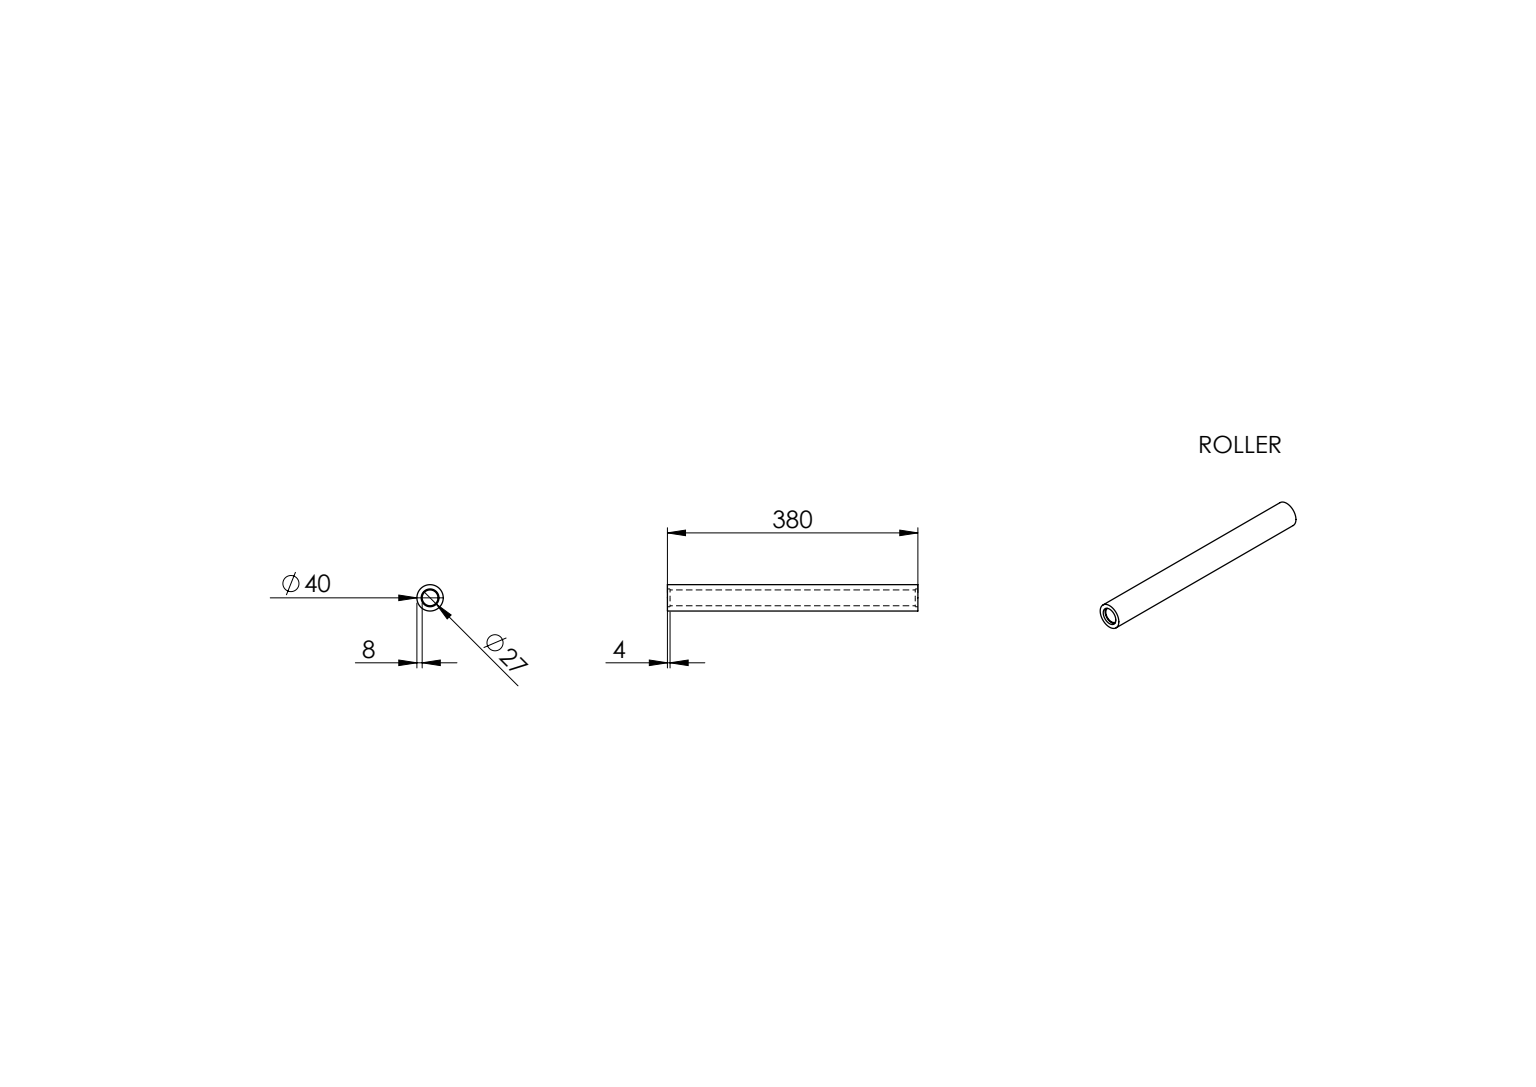
ISO-10303-21;
HEADER;
FILE_DESCRIPTION (('STEP AP214'),
    '1' );
FILE_NAME ('roller.step',
    '2026-10-24T13:33:06',
    ( '' ),
    ( '' ),
    'SwSTEP 2.0',
    'SolidWorks 2026',
    '' );
FILE_SCHEMA (( 'AUTOMOTIVE_DESIGN' ));
ENDSEC;

DATA;
#56=DIRECTION ( 'NONE',  ( 1.000000000000000000, 0.000000000000000000, 0.000000000000000000 ) ) ;
#77=FACE_OUTER_BOUND ( 'NONE', #3479, .T. ) ;
#137=ORIENTED_EDGE ( 'NONE', *, *, #8244, .F. ) ;
#171=CIRCLE ( 'NONE', #3238, 20.00000000000000000 ) ;
#191=VERTEX_POINT ( 'NONE', #7546 ) ;
#269=LINE ( 'NONE', #13422, #9164 ) ;
#370=DIRECTION ( 'NONE',  ( -1.000000000000000000, 0.000000000000000000, 0.000000000000000000 ) ) ;
#456=ORIENTED_EDGE ( 'NONE', *, *, #9949, .T. ) ;
#491=( GEOMETRIC_REPRESENTATION_CONTEXT ( 3 ) GLOBAL_UNCERTAINTY_ASSIGNED_CONTEXT ( ( #7550 ) ) GLOBAL_UNIT_ASSIGNED_CONTEXT ( ( #9395, #10194, #4976 ) ) REPRESENTATION_CONTEXT ( 'NONE', 'WORKASPACE' ) );
#495=EDGE_LOOP ( 'NONE', ( #2805, #3128, #6532, #2703 ) ) ;
#498=VERTEX_POINT ( 'NONE', #10666 ) ;
#571=DIRECTION ( 'NONE',  ( -0.000000000000000000, -0.000000000000000000, -1.000000000000000000 ) ) ;
#599=CARTESIAN_POINT ( 'NONE',  ( 0.000000000000000000, 0.000000000000000000, 186.0000000000000000 ) ) ;
#655=CARTESIAN_POINT ( 'NONE',  ( 0.000000000000000000, 0.000000000000000000, 186.0000000000000000 ) ) ;
#810=DIRECTION ( 'NONE',  ( 1.000000000000000000, 0.000000000000000000, 0.000000000000000000 ) ) ;
#928=CIRCLE ( 'NONE', #9057, 13.50000000000000000 ) ;
#944=ORIENTED_EDGE ( 'NONE', *, *, #12577, .T. ) ;
#1054=ADVANCED_BREP_SHAPE_REPRESENTATION ( '', ( #8362, #14039 ), #4925 ) ;
#1097=AXIS2_PLACEMENT_3D ( 'NONE', #1465, #6917, #7059 ) ;
#1124=AXIS2_PLACEMENT_3D ( 'NONE', #13971, #12956, #3031 ) ;
#1240=DIRECTION ( 'NONE',  ( 0.000000000000000000, 0.000000000000000000, 1.000000000000000000 ) ) ;
#1273=CARTESIAN_POINT ( 'NONE',  ( -13.50000000000000000, 1.653273178848926867E-15, 186.0000000000000000 ) ) ;
#1296=ORIENTED_EDGE ( 'NONE', *, *, #6936, .T. ) ;
#1318=AXIS2_PLACEMENT_3D ( 'NONE', #6760, #2269, #6696 ) ;
#1331=EDGE_CURVE ( 'NONE', #11674, #5306, #12710, .T. ) ;
#1464=FACE_OUTER_BOUND ( 'NONE', #495, .T. ) ;
#1465=CARTESIAN_POINT ( 'NONE',  ( 0.000000000000000000, 0.000000000000000000, 190.0000000000000000 ) ) ;
#1505=EDGE_LOOP ( 'NONE', ( #3985, #10939 ) ) ;
#1537=CARTESIAN_POINT ( 'NONE',  ( 0.000000000000000000, 0.000000000000000000, -186.0000000000000000 ) ) ;
#1589=( LENGTH_UNIT ( ) NAMED_UNIT ( * ) SI_UNIT ( .MILLI., .METRE. ) );
#1620=SURFACE_STYLE_FILL_AREA ( #2512 ) ;
#1624=CARTESIAN_POINT ( 'NONE',  ( 0.000000000000000000, 0.000000000000000000, -186.0000000000000000 ) ) ;
#1684=UNCERTAINTY_MEASURE_WITH_UNIT (LENGTH_MEASURE( 1.000000000000000082E-05 ), #1589, 'distance_accuracy_value', 'NONE');
#1739=PRODUCT_CONTEXT ( 'NONE', #11106, 'mechanical' ) ;
#1792=ADVANCED_FACE ( 'NONE', ( #5012 ), #10742, .F. ) ;
#1814=( NAMED_UNIT ( * ) PLANE_ANGLE_UNIT ( ) SI_UNIT ( $, .RADIAN. ) );
#1924=APPLICATION_CONTEXT ( 'automotive_design' ) ;
#1936=EDGE_LOOP ( 'NONE', ( #2189, #10105 ) ) ;
#1948=EDGE_CURVE ( 'NONE', #3491, #8933, #13191, .T. ) ;
#1979=CARTESIAN_POINT ( 'NONE',  ( 12.00000000000000000, 1.469576158976823947E-15, 186.0000000000000000 ) ) ;
#2027=AXIS2_PLACEMENT_3D ( 'NONE', #10148, #6674, #12325 ) ;
#2063=CYLINDRICAL_SURFACE ( 'NONE', #8959, 13.50000000000000000 ) ;
#2070=CIRCLE ( 'NONE', #12034, 13.50000000000000000 ) ;
#2075=ORIENTED_EDGE ( 'NONE', *, *, #12736, .F. ) ;
#2081=AXIS2_PLACEMENT_3D ( 'NONE', #6577, #11081, #6714 ) ;
#2151=EDGE_CURVE ( 'NONE', #4585, #8933, #7405, .T. ) ;
#2189=ORIENTED_EDGE ( 'NONE', *, *, #13813, .F. ) ;
#2217=ADVANCED_FACE ( 'NONE', ( #13247, #6644 ), #8752, .T. ) ;
#2269=DIRECTION ( 'NONE',  ( 0.000000000000000000, 0.000000000000000000, 1.000000000000000000 ) ) ;
#2309=DIRECTION ( 'NONE',  ( -0.000000000000000000, -0.000000000000000000, 1.000000000000000000 ) ) ;
#2414=DIRECTION ( 'NONE',  ( 1.000000000000000000, 0.000000000000000000, 0.000000000000000000 ) ) ;
#2437=VERTEX_POINT ( 'NONE', #8958 ) ;
#2460=DIRECTION ( 'NONE',  ( 0.000000000000000000, 0.000000000000000000, 1.000000000000000000 ) ) ;
#2512=FILL_AREA_STYLE ('',( #5766 ) ) ;
#2703=ORIENTED_EDGE ( 'NONE', *, *, #3672, .T. ) ;
#2712=ORIENTED_EDGE ( 'NONE', *, *, #6511, .T. ) ;
#2727=SHAPE_REPRESENTATION_RELATIONSHIP ( 'NONE' , 'NONE' ,  #11637, #1054 ) ;
#2755=ORIENTED_EDGE ( 'NONE', *, *, #4202, .T. ) ;
#2759=ORIENTED_EDGE ( 'NONE', *, *, #3672, .F. ) ;
#2783=CARTESIAN_POINT ( 'NONE',  ( -13.50000000000000000, 0.000000000000000000, -186.0000000000000000 ) ) ;
#2794=CARTESIAN_POINT ( 'NONE',  ( -13.50000000000000000, 0.000000000000000000, -190.0000000000000000 ) ) ;
#2805=ORIENTED_EDGE ( 'NONE', *, *, #11204, .F. ) ;
#2810=VECTOR ( 'NONE', #7862, 1000.000000000000000 ) ;
#2822=( NAMED_UNIT ( * ) PLANE_ANGLE_UNIT ( ) SI_UNIT ( $, .RADIAN. ) );
#2862=CYLINDRICAL_SURFACE ( 'NONE', #13359, 13.50000000000000000 ) ;
#2866=DIRECTION ( 'NONE',  ( 0.000000000000000000, 0.000000000000000000, -1.000000000000000000 ) ) ;
#2910=CARTESIAN_POINT ( 'NONE',  ( -20.00000000000000000, 0.000000000000000000, -190.0000000000000000 ) ) ;
#3006=FACE_BOUND ( 'NONE', #5352, .T. ) ;
#3031=DIRECTION ( 'NONE',  ( -1.000000000000000000, 0.000000000000000000, 0.000000000000000000 ) ) ;
#3101=FACE_OUTER_BOUND ( 'NONE', #12272, .T. ) ;
#3107=DIRECTION ( 'NONE',  ( 1.000000000000000000, 0.000000000000000000, 0.000000000000000000 ) ) ;
#3119=CARTESIAN_POINT ( 'NONE',  ( -20.00000000000000000, 0.000000000000000000, 190.0000000000000000 ) ) ;
#3128=ORIENTED_EDGE ( 'NONE', *, *, #4828, .F. ) ;
#3226=CARTESIAN_POINT ( 'NONE',  ( 0.000000000000000000, 0.000000000000000000, 190.0000000000000000 ) ) ;
#3238=AXIS2_PLACEMENT_3D ( 'NONE', #7957, #2460, #6956 ) ;
#3276=CARTESIAN_POINT ( 'NONE',  ( 20.00000000000000000, 2.449293598294706513E-15, 190.0000000000000000 ) ) ;
#3357=ADVANCED_FACE ( 'NONE', ( #77 ), #5296, .F. ) ;
#3367=FACE_OUTER_BOUND ( 'NONE', #7390, .T. ) ;
#3479=EDGE_LOOP ( 'NONE', ( #3545, #1296, #9689, #9133 ) ) ;
#3491=VERTEX_POINT ( 'NONE', #9320 ) ;
#3512=CARTESIAN_POINT ( 'NONE',  ( 0.000000000000000000, 0.000000000000000000, 186.0000000000000000 ) ) ;
#3520=DIRECTION ( 'NONE',  ( 1.000000000000000000, 0.000000000000000000, 0.000000000000000000 ) ) ;
#3539=ADVANCED_FACE ( 'NONE', ( #11426 ), #6123, .T. ) ;
#3545=ORIENTED_EDGE ( 'NONE', *, *, #5646, .T. ) ;
#3555=DIRECTION ( 'NONE',  ( -1.000000000000000000, 0.000000000000000000, 0.000000000000000000 ) ) ;
#3571=DIRECTION ( 'NONE',  ( 1.000000000000000000, 0.000000000000000000, 0.000000000000000000 ) ) ;
#3581=VERTEX_POINT ( 'NONE', #1979 ) ;
#3622=FACE_OUTER_BOUND ( 'NONE', #11623, .T. ) ;
#3642=CIRCLE ( 'NONE', #1318, 20.00000000000000000 ) ;
#3672=EDGE_CURVE ( 'NONE', #191, #8653, #928, .T. ) ;
#3744=AXIS2_PLACEMENT_3D ( 'NONE', #5000, #13836, #6082 ) ;
#3761=ORIENTED_EDGE ( 'NONE', *, *, #5646, .F. ) ;
#3785=ORIENTED_EDGE ( 'NONE', *, *, #12600, .F. ) ;
#3841=CARTESIAN_POINT ( 'NONE',  ( 0.000000000000000000, 0.000000000000000000, 190.0000000000000000 ) ) ;
#3885=ORIENTED_EDGE ( 'NONE', *, *, #6936, .F. ) ;
#3927=DIRECTION ( 'NONE',  ( 0.000000000000000000, 0.000000000000000000, 1.000000000000000000 ) ) ;
#3935=AXIS2_PLACEMENT_3D ( 'NONE', #7654, #9770, #12149 ) ;
#3952=DIRECTION ( 'NONE',  ( -0.000000000000000000, -0.000000000000000000, -1.000000000000000000 ) ) ;
#3985=ORIENTED_EDGE ( 'NONE', *, *, #8012, .F. ) ;
#4003=STYLED_ITEM ( 'NONE', ( #12442 ), #1054 ) ;
#4123=CIRCLE ( 'NONE', #5473, 20.00000000000000000 ) ;
#4195=EDGE_LOOP ( 'NONE', ( #2759, #5420 ) ) ;
#4202=EDGE_CURVE ( 'NONE', #8845, #7342, #171, .T. ) ;
#4203=ADVANCED_FACE ( 'NONE', ( #3622 ), #10363, .T. ) ;
#4210=CARTESIAN_POINT ( 'NONE',  ( -12.00000000000000000, 0.000000000000000000, 190.0000000000000000 ) ) ;
#4380=ORIENTED_EDGE ( 'NONE', *, *, #9949, .F. ) ;
#4448=LINE ( 'NONE', #8868, #13591 ) ;
#4513=ORIENTED_EDGE ( 'NONE', *, *, #11633, .T. ) ;
#4516=FACE_BOUND ( 'NONE', #1505, .T. ) ;
#4567=CARTESIAN_POINT ( 'NONE',  ( 0.000000000000000000, 0.000000000000000000, 186.0000000000000000 ) ) ;
#4585=VERTEX_POINT ( 'NONE', #10949 ) ;
#4644=VECTOR ( 'NONE', #13052, 1000.000000000000000 ) ;
#4647=CARTESIAN_POINT ( 'NONE',  ( 20.00000000000000000, 2.449293598294706513E-15, -190.0000000000000000 ) ) ;
#4755=DIRECTION ( 'NONE',  ( -1.000000000000000000, 0.000000000000000000, 0.000000000000000000 ) ) ;
#4762=FACE_OUTER_BOUND ( 'NONE', #8447, .T. ) ;
#4783=CYLINDRICAL_SURFACE ( 'NONE', #6286, 13.50000000000000000 ) ;
#4804=DIRECTION ( 'NONE',  ( -0.000000000000000000, -0.000000000000000000, 1.000000000000000000 ) ) ;
#4816=CIRCLE ( 'NONE', #2027, 13.50000000000000000 ) ;
#4828=EDGE_CURVE ( 'NONE', #2437, #12064, #2070, .T. ) ;
#4878=ORIENTED_EDGE ( 'NONE', *, *, #11204, .T. ) ;
#4925=( GEOMETRIC_REPRESENTATION_CONTEXT ( 3 ) GLOBAL_UNCERTAINTY_ASSIGNED_CONTEXT ( ( #11924 ) ) GLOBAL_UNIT_ASSIGNED_CONTEXT ( ( #8462, #2822, #9489 ) ) REPRESENTATION_CONTEXT ( 'NONE', 'WORKASPACE' ) );
#4976=( NAMED_UNIT ( * ) SI_UNIT ( $, .STERADIAN. ) SOLID_ANGLE_UNIT ( ) );
#4992=EDGE_CURVE ( 'NONE', #498, #11674, #12043, .T. ) ;
#5000=CARTESIAN_POINT ( 'NONE',  ( 0.000000000000000000, 0.000000000000000000, 186.0000000000000000 ) ) ;
#5012=FACE_OUTER_BOUND ( 'NONE', #13790, .T. ) ;
#5048=AXIS2_PLACEMENT_3D ( 'NONE', #12411, #4804, #3571 ) ;
#5077=DIRECTION ( 'NONE',  ( 1.000000000000000000, 0.000000000000000000, 0.000000000000000000 ) ) ;
#5296=CYLINDRICAL_SURFACE ( 'NONE', #6955, 12.00000000000000000 ) ;
#5299=AXIS2_PLACEMENT_3D ( 'NONE', #1624, #8084, #370 ) ;
#5306=VERTEX_POINT ( 'NONE', #2794 ) ;
#5352=EDGE_LOOP ( 'NONE', ( #2712, #8869 ) ) ;
#5385=VECTOR ( 'NONE', #571, 1000.000000000000000 ) ;
#5394=PLANE ( 'NONE',  #10352 ) ;
#5420=ORIENTED_EDGE ( 'NONE', *, *, #8564, .F. ) ;
#5473=AXIS2_PLACEMENT_3D ( 'NONE', #10605, #3927, #6243 ) ;
#5487=AXIS2_PLACEMENT_3D ( 'NONE', #13439, #9021, #3520 ) ;
#5493=VECTOR ( 'NONE', #5601, 1000.000000000000000 ) ;
#5591=ORIENTED_EDGE ( 'NONE', *, *, #7420, .F. ) ;
#5595=PRODUCT_DEFINITION ( 'UNKNOWN', '', #8389, #11885 ) ;
#5601=DIRECTION ( 'NONE',  ( -0.000000000000000000, -0.000000000000000000, -1.000000000000000000 ) ) ;
#5636=LINE ( 'NONE', #7935, #2810 ) ;
#5646=EDGE_CURVE ( 'NONE', #3491, #3581, #13595, .T. ) ;
#5766=FILL_AREA_STYLE_COLOUR ( '', #10253 ) ;
#5773=CARTESIAN_POINT ( 'NONE',  ( -12.00000000000000000, 0.000000000000000000, -186.0000000000000000 ) ) ;
#5880=LINE ( 'NONE', #13419, #11078 ) ;
#6082=DIRECTION ( 'NONE',  ( 1.000000000000000000, 0.000000000000000000, 0.000000000000000000 ) ) ;
#6123=CYLINDRICAL_SURFACE ( 'NONE', #12305, 20.00000000000000000 ) ;
#6243=DIRECTION ( 'NONE',  ( 1.000000000000000000, 0.000000000000000000, 0.000000000000000000 ) ) ;
#6282=VERTEX_POINT ( 'NONE', #4647 ) ;
#6286=AXIS2_PLACEMENT_3D ( 'NONE', #13335, #9203, #3555 ) ;
#6324=AXIS2_PLACEMENT_3D ( 'NONE', #3841, #8257, #13916 ) ;
#6340=FACE_OUTER_BOUND ( 'NONE', #1936, .T. ) ;
#6347=DIRECTION ( 'NONE',  ( 0.000000000000000000, 0.000000000000000000, 1.000000000000000000 ) ) ;
#6511=EDGE_CURVE ( 'NONE', #5306, #7372, #8732, .T. ) ;
#6532=ORIENTED_EDGE ( 'NONE', *, *, #12600, .T. ) ;
#6567=ADVANCED_FACE ( 'NONE', ( #1464 ), #2862, .F. ) ;
#6577=CARTESIAN_POINT ( 'NONE',  ( 0.000000000000000000, 0.000000000000000000, 186.0000000000000000 ) ) ;
#6616=LINE ( 'NONE', #12065, #5493 ) ;
#6639=CARTESIAN_POINT ( 'NONE',  ( 0.000000000000000000, 0.000000000000000000, 190.0000000000000000 ) ) ;
#6644=FACE_OUTER_BOUND ( 'NONE', #11694, .T. ) ;
#6650=CIRCLE ( 'NONE', #5048, 13.50000000000000000 ) ;
#6666=DIRECTION ( 'NONE',  ( -0.000000000000000000, -0.000000000000000000, 1.000000000000000000 ) ) ;
#6674=DIRECTION ( 'NONE',  ( 0.000000000000000000, 0.000000000000000000, 1.000000000000000000 ) ) ;
#6696=DIRECTION ( 'NONE',  ( 1.000000000000000000, 0.000000000000000000, 0.000000000000000000 ) ) ;
#6714=DIRECTION ( 'NONE',  ( 1.000000000000000000, 0.000000000000000000, -0.000000000000000000 ) ) ;
#6729=AXIS2_PLACEMENT_3D ( 'NONE', #10069, #6666, #8915 ) ;
#6750=EDGE_LOOP ( 'NONE', ( #11100, #13181, #13851, #6805 ) ) ;
#6760=CARTESIAN_POINT ( 'NONE',  ( 0.000000000000000000, 0.000000000000000000, -190.0000000000000000 ) ) ;
#6805=ORIENTED_EDGE ( 'NONE', *, *, #12577, .F. ) ;
#6880=CIRCLE ( 'NONE', #7111, 12.00000000000000000 ) ;
#6917=DIRECTION ( 'NONE',  ( 0.000000000000000000, 0.000000000000000000, 1.000000000000000000 ) ) ;
#6936=EDGE_CURVE ( 'NONE', #3581, #4585, #269, .T. ) ;
#6955=AXIS2_PLACEMENT_3D ( 'NONE', #6639, #9025, #9102 ) ;
#6956=DIRECTION ( 'NONE',  ( 1.000000000000000000, 0.000000000000000000, 0.000000000000000000 ) ) ;
#7059=DIRECTION ( 'NONE',  ( 1.000000000000000000, 0.000000000000000000, 0.000000000000000000 ) ) ;
#7111=AXIS2_PLACEMENT_3D ( 'NONE', #1537, #2866, #8210 ) ;
#7115=( NAMED_UNIT ( * ) SI_UNIT ( $, .STERADIAN. ) SOLID_ANGLE_UNIT ( ) );
#7198=DIRECTION ( 'NONE',  ( 1.000000000000000000, 0.000000000000000000, 0.000000000000000000 ) ) ;
#7222=VECTOR ( 'NONE', #2309, 1000.000000000000000 ) ;
#7250=VERTEX_POINT ( 'NONE', #2910 ) ;
#7262=SHAPE_DEFINITION_REPRESENTATION ( #8896, #11637 ) ;
#7293=DIRECTION ( 'NONE',  ( 0.000000000000000000, 0.000000000000000000, 1.000000000000000000 ) ) ;
#7342=VERTEX_POINT ( 'NONE', #3276 ) ;
#7344=AXIS2_PLACEMENT_3D ( 'NONE', #14226, #10032, #56 ) ;
#7364=CIRCLE ( 'NONE', #1097, 20.00000000000000000 ) ;
#7372=VERTEX_POINT ( 'NONE', #9940 ) ;
#7390=EDGE_LOOP ( 'NONE', ( #8455, #12832 ) ) ;
#7405=CIRCLE ( 'NONE', #1124, 12.00000000000000000 ) ;
#7420=EDGE_CURVE ( 'NONE', #12064, #2437, #7557, .T. ) ;
#7422=DIRECTION ( 'NONE',  ( 1.000000000000000000, 0.000000000000000000, -0.000000000000000000 ) ) ;
#7546=CARTESIAN_POINT ( 'NONE',  ( 13.50000000000000000, 0.000000000000000000, 190.0000000000000000 ) ) ;
#7550=UNCERTAINTY_MEASURE_WITH_UNIT (LENGTH_MEASURE( 1.000000000000000082E-05 ), #9395, 'distance_accuracy_value', 'NONE');
#7557=CIRCLE ( 'NONE', #10331, 13.50000000000000000 ) ;
#7627=DIRECTION ( 'NONE',  ( -0.000000000000000000, -0.000000000000000000, 1.000000000000000000 ) ) ;
#7654=CARTESIAN_POINT ( 'NONE',  ( 0.000000000000000000, 0.000000000000000000, -186.0000000000000000 ) ) ;
#7744=LINE ( 'NONE', #1273, #7222 ) ;
#7862=DIRECTION ( 'NONE',  ( -0.000000000000000000, -0.000000000000000000, -1.000000000000000000 ) ) ;
#7901=DIRECTION ( 'NONE',  ( -0.000000000000000000, -0.000000000000000000, -1.000000000000000000 ) ) ;
#7935=CARTESIAN_POINT ( 'NONE',  ( 13.50000000000000000, 1.653273178848926867E-15, -186.0000000000000000 ) ) ;
#7957=CARTESIAN_POINT ( 'NONE',  ( 0.000000000000000000, 0.000000000000000000, 190.0000000000000000 ) ) ;
#8012=EDGE_CURVE ( 'NONE', #8933, #4585, #6880, .T. ) ;
#8084=DIRECTION ( 'NONE',  ( -0.000000000000000000, -0.000000000000000000, -1.000000000000000000 ) ) ;
#8210=DIRECTION ( 'NONE',  ( -1.000000000000000000, 0.000000000000000000, 0.000000000000000000 ) ) ;
#8244=EDGE_CURVE ( 'NONE', #7372, #5306, #6650, .T. ) ;
#8257=DIRECTION ( 'NONE',  ( -0.000000000000000000, -0.000000000000000000, -1.000000000000000000 ) ) ;
#8362=MANIFOLD_SOLID_BREP ( 'Mirror1', #9140 ) ;
#8389=PRODUCT_DEFINITION_FORMATION_WITH_SPECIFIED_SOURCE ( 'ANY', '', #13394, .NOT_KNOWN. ) ;
#8447=EDGE_LOOP ( 'NONE', ( #12356, #4513, #11568, #10836 ) ) ;
#8455=ORIENTED_EDGE ( 'NONE', *, *, #11116, .F. ) ;
#8462=( LENGTH_UNIT ( ) NAMED_UNIT ( * ) SI_UNIT ( .MILLI., .METRE. ) );
#8564=EDGE_CURVE ( 'NONE', #8653, #191, #4816, .T. ) ;
#8653=VERTEX_POINT ( 'NONE', #13536 ) ;
#8732=CIRCLE ( 'NONE', #5487, 13.50000000000000000 ) ;
#8752=PLANE ( 'NONE',  #2081 ) ;
#8796=DIRECTION ( 'NONE',  ( 0.000000000000000000, 0.000000000000000000, 1.000000000000000000 ) ) ;
#8845=VERTEX_POINT ( 'NONE', #3119 ) ;
#8868=CARTESIAN_POINT ( 'NONE',  ( 13.50000000000000000, 0.000000000000000000, 186.0000000000000000 ) ) ;
#8869=ORIENTED_EDGE ( 'NONE', *, *, #8244, .T. ) ;
#8870=DIRECTION ( 'NONE',  ( -0.000000000000000000, -0.000000000000000000, -1.000000000000000000 ) ) ;
#8896=PRODUCT_DEFINITION_SHAPE ( 'NONE', 'NONE',  #5595 ) ;
#8915=DIRECTION ( 'NONE',  ( 1.000000000000000000, 0.000000000000000000, 0.000000000000000000 ) ) ;
#8918=DIRECTION ( 'NONE',  ( 0.000000000000000000, 0.000000000000000000, 1.000000000000000000 ) ) ;
#8933=VERTEX_POINT ( 'NONE', #5773 ) ;
#8958=CARTESIAN_POINT ( 'NONE',  ( 13.50000000000000000, 0.000000000000000000, 186.0000000000000000 ) ) ;
#8959=AXIS2_PLACEMENT_3D ( 'NONE', #9546, #13962, #810 ) ;
#8967=EDGE_LOOP ( 'NONE', ( #2755, #10976 ) ) ;
#9021=DIRECTION ( 'NONE',  ( -0.000000000000000000, -0.000000000000000000, 1.000000000000000000 ) ) ;
#9025=DIRECTION ( 'NONE',  ( -0.000000000000000000, -0.000000000000000000, -1.000000000000000000 ) ) ;
#9057=AXIS2_PLACEMENT_3D ( 'NONE', #12939, #6347, #9755 ) ;
#9079=CIRCLE ( 'NONE', #6729, 13.50000000000000000 ) ;
#9102=DIRECTION ( 'NONE',  ( -1.000000000000000000, 0.000000000000000000, 0.000000000000000000 ) ) ;
#9103=CARTESIAN_POINT ( 'NONE',  ( -13.50000000000000000, 0.000000000000000000, -186.0000000000000000 ) ) ;
#9133=ORIENTED_EDGE ( 'NONE', *, *, #1948, .F. ) ;
#9140=CLOSED_SHELL ( 'NONE', ( #13154, #11889, #3539, #3357, #1792, #12529, #12429, #4203, #6567, #2217, #9916, #12604 ) ) ;
#9164=VECTOR ( 'NONE', #8870, 1000.000000000000000 ) ;
#9175=CYLINDRICAL_SURFACE ( 'NONE', #5299, 13.50000000000000000 ) ;
#9203=DIRECTION ( 'NONE',  ( -0.000000000000000000, -0.000000000000000000, -1.000000000000000000 ) ) ;
#9320=CARTESIAN_POINT ( 'NONE',  ( -12.00000000000000000, 0.000000000000000000, 186.0000000000000000 ) ) ;
#9395=( LENGTH_UNIT ( ) NAMED_UNIT ( * ) SI_UNIT ( .MILLI., .METRE. ) );
#9418=DIRECTION ( 'NONE',  ( 0.000000000000000000, 0.000000000000000000, 1.000000000000000000 ) ) ;
#9486=ORIENTED_EDGE ( 'NONE', *, *, #8012, .T. ) ;
#9489=( NAMED_UNIT ( * ) SI_UNIT ( $, .STERADIAN. ) SOLID_ANGLE_UNIT ( ) );
#9546=CARTESIAN_POINT ( 'NONE',  ( 0.000000000000000000, 0.000000000000000000, 186.0000000000000000 ) ) ;
#9689=ORIENTED_EDGE ( 'NONE', *, *, #2151, .T. ) ;
#9748=PLANE ( 'NONE',  #12439 ) ;
#9755=DIRECTION ( 'NONE',  ( 1.000000000000000000, 0.000000000000000000, 0.000000000000000000 ) ) ;
#9770=DIRECTION ( 'NONE',  ( -0.000000000000000000, -0.000000000000000000, 1.000000000000000000 ) ) ;
#9916=ADVANCED_FACE ( 'NONE', ( #13475 ), #4783, .F. ) ;
#9940=CARTESIAN_POINT ( 'NONE',  ( 13.50000000000000000, 1.653273178848926867E-15, -190.0000000000000000 ) ) ;
#9949=EDGE_CURVE ( 'NONE', #3581, #3491, #10004, .T. ) ;
#10004=CIRCLE ( 'NONE', #3744, 12.00000000000000000 ) ;
#10032=DIRECTION ( 'NONE',  ( 0.000000000000000000, 0.000000000000000000, -1.000000000000000000 ) ) ;
#10069=CARTESIAN_POINT ( 'NONE',  ( 0.000000000000000000, 0.000000000000000000, -186.0000000000000000 ) ) ;
#10105=ORIENTED_EDGE ( 'NONE', *, *, #14017, .F. ) ;
#10148=CARTESIAN_POINT ( 'NONE',  ( 0.000000000000000000, 0.000000000000000000, 190.0000000000000000 ) ) ;
#10194=( NAMED_UNIT ( * ) PLANE_ANGLE_UNIT ( ) SI_UNIT ( $, .RADIAN. ) );
#10253=COLOUR_RGB ( '',0.8941176470588234615, 0.8941176470588234615, 0.8941176470588234615 ) ;
#10331=AXIS2_PLACEMENT_3D ( 'NONE', #4567, #8918, #13196 ) ;
#10352=AXIS2_PLACEMENT_3D ( 'NONE', #3226, #8796, #13073 ) ;
#10363=CYLINDRICAL_SURFACE ( 'NONE', #14105, 20.00000000000000000 ) ;
#10508=CARTESIAN_POINT ( 'NONE',  ( 0.000000000000000000, 0.000000000000000000, 0.000000000000000000 ) ) ;
#10605=CARTESIAN_POINT ( 'NONE',  ( 0.000000000000000000, 0.000000000000000000, -190.0000000000000000 ) ) ;
#10666=CARTESIAN_POINT ( 'NONE',  ( 13.50000000000000000, 1.653273178848926867E-15, -186.0000000000000000 ) ) ;
#10694=DIRECTION ( 'NONE',  ( 0.000000000000000000, 0.000000000000000000, 1.000000000000000000 ) ) ;
#10742=CYLINDRICAL_SURFACE ( 'NONE', #6324, 12.00000000000000000 ) ;
#10836=ORIENTED_EDGE ( 'NONE', *, *, #1331, .F. ) ;
#10906=PLANE ( 'NONE',  #7344 ) ;
#10939=ORIENTED_EDGE ( 'NONE', *, *, #2151, .F. ) ;
#10949=CARTESIAN_POINT ( 'NONE',  ( 12.00000000000000000, 1.469576158976823947E-15, -186.0000000000000000 ) ) ;
#10962=EDGE_LOOP ( 'NONE', ( #3761, #4380 ) ) ;
#10976=ORIENTED_EDGE ( 'NONE', *, *, #13401, .T. ) ;
#11078=VECTOR ( 'NONE', #7901, 1000.000000000000000 ) ;
#11081=DIRECTION ( 'NONE',  ( 0.000000000000000000, 0.000000000000000000, 1.000000000000000000 ) ) ;
#11100=ORIENTED_EDGE ( 'NONE', *, *, #13401, .F. ) ;
#11106=APPLICATION_CONTEXT ( 'automotive_design' ) ;
#11116=EDGE_CURVE ( 'NONE', #11674, #498, #9079, .T. ) ;
#11204=EDGE_CURVE ( 'NONE', #12064, #8653, #7744, .T. ) ;
#11319=DIRECTION ( 'NONE',  ( -0.000000000000000000, -0.000000000000000000, -1.000000000000000000 ) ) ;
#11340=EDGE_LOOP ( 'NONE', ( #11480, #13941, #14030, #137 ) ) ;
#11358=SURFACE_STYLE_USAGE ( .BOTH. , #13740 ) ;
#11426=FACE_OUTER_BOUND ( 'NONE', #6750, .T. ) ;
#11480=ORIENTED_EDGE ( 'NONE', *, *, #11633, .F. ) ;
#11521=AXIS2_PLACEMENT_3D ( 'NONE', #3512, #1240, #2414 ) ;
#11568=ORIENTED_EDGE ( 'NONE', *, *, #6511, .F. ) ;
#11623=EDGE_LOOP ( 'NONE', ( #2075, #13914, #944, #12733 ) ) ;
#11633=EDGE_CURVE ( 'NONE', #498, #7372, #5636, .T. ) ;
#11637=SHAPE_REPRESENTATION ( 'roller', ( #14039 ), #4925 ) ;
#11674=VERTEX_POINT ( 'NONE', #9103 ) ;
#11679=ORIENTED_EDGE ( 'NONE', *, *, #7420, .T. ) ;
#11694=EDGE_LOOP ( 'NONE', ( #11711, #11679 ) ) ;
#11711=ORIENTED_EDGE ( 'NONE', *, *, #4828, .T. ) ;
#11885=PRODUCT_DEFINITION_CONTEXT ( 'detailed design', #1924, 'design' ) ;
#11889=ADVANCED_FACE ( 'NONE', ( #3101 ), #2063, .F. ) ;
#11924=UNCERTAINTY_MEASURE_WITH_UNIT (LENGTH_MEASURE( 1.000000000000000082E-05 ), #8462, 'distance_accuracy_value', 'NONE');
#12034=AXIS2_PLACEMENT_3D ( 'NONE', #599, #7293, #3107 ) ;
#12043=CIRCLE ( 'NONE', #3935, 13.50000000000000000 ) ;
#12064=VERTEX_POINT ( 'NONE', #12216 ) ;
#12065=CARTESIAN_POINT ( 'NONE',  ( -20.00000000000000000, 0.000000000000000000, 190.0000000000000000 ) ) ;
#12149=DIRECTION ( 'NONE',  ( 1.000000000000000000, 0.000000000000000000, 0.000000000000000000 ) ) ;
#12216=CARTESIAN_POINT ( 'NONE',  ( -13.50000000000000000, 1.653273178848926867E-15, 186.0000000000000000 ) ) ;
#12272=EDGE_LOOP ( 'NONE', ( #5591, #4878, #13037, #3785 ) ) ;
#12274=FACE_OUTER_BOUND ( 'NONE', #8967, .T. ) ;
#12305=AXIS2_PLACEMENT_3D ( 'NONE', #13875, #3952, #4755 ) ;
#12325=DIRECTION ( 'NONE',  ( 1.000000000000000000, 0.000000000000000000, 0.000000000000000000 ) ) ;
#12356=ORIENTED_EDGE ( 'NONE', *, *, #11116, .T. ) ;
#12411=CARTESIAN_POINT ( 'NONE',  ( 0.000000000000000000, 0.000000000000000000, -190.0000000000000000 ) ) ;
#12429=ADVANCED_FACE ( 'NONE', ( #3006, #6340 ), #9748, .F. ) ;
#12439=AXIS2_PLACEMENT_3D ( 'NONE', #13942, #10694, #7422 ) ;
#12442=PRESENTATION_STYLE_ASSIGNMENT (( #11358 ) ) ;
#12463=ORIENTED_EDGE ( 'NONE', *, *, #1948, .T. ) ;
#12529=ADVANCED_FACE ( 'NONE', ( #13348, #12274 ), #5394, .T. ) ;
#12545=CARTESIAN_POINT ( 'NONE',  ( 0.000000000000000000, 0.000000000000000000, 190.0000000000000000 ) ) ;
#12577=EDGE_CURVE ( 'NONE', #8845, #7250, #6616, .T. ) ;
#12600=EDGE_CURVE ( 'NONE', #2437, #191, #4448, .T. ) ;
#12604=ADVANCED_FACE ( 'NONE', ( #4516, #3367 ), #10906, .T. ) ;
#12609=DIRECTION ( 'NONE',  ( -1.000000000000000000, 0.000000000000000000, 0.000000000000000000 ) ) ;
#12667=STYLED_ITEM('',(#14403),#8362);
#12679=( GEOMETRIC_REPRESENTATION_CONTEXT ( 3 ) GLOBAL_UNCERTAINTY_ASSIGNED_CONTEXT ( ( #1684 ) ) GLOBAL_UNIT_ASSIGNED_CONTEXT ( ( #1589, #1814, #7115 ) ) REPRESENTATION_CONTEXT ( 'NONE', 'WORKASPACE' ) );
#12710=LINE ( 'NONE', #2783, #5385 ) ;
#12733=ORIENTED_EDGE ( 'NONE', *, *, #13813, .T. ) ;
#12736=EDGE_CURVE ( 'NONE', #7342, #6282, #5880, .T. ) ;
#12832=ORIENTED_EDGE ( 'NONE', *, *, #4992, .F. ) ;
#12939=CARTESIAN_POINT ( 'NONE',  ( 0.000000000000000000, 0.000000000000000000, 190.0000000000000000 ) ) ;
#12956=DIRECTION ( 'NONE',  ( 0.000000000000000000, 0.000000000000000000, -1.000000000000000000 ) ) ;
#13037=ORIENTED_EDGE ( 'NONE', *, *, #8564, .T. ) ;
#13052=DIRECTION ( 'NONE',  ( -0.000000000000000000, -0.000000000000000000, -1.000000000000000000 ) ) ;
#13073=DIRECTION ( 'NONE',  ( 1.000000000000000000, 0.000000000000000000, -0.000000000000000000 ) ) ;
#13154=ADVANCED_FACE ( 'NONE', ( #4762 ), #9175, .F. ) ;
#13181=ORIENTED_EDGE ( 'NONE', *, *, #12736, .T. ) ;
#13191=LINE ( 'NONE', #4210, #4644 ) ;
#13196=DIRECTION ( 'NONE',  ( 1.000000000000000000, 0.000000000000000000, 0.000000000000000000 ) ) ;
#13247=FACE_BOUND ( 'NONE', #10962, .T. ) ;
#13335=CARTESIAN_POINT ( 'NONE',  ( 0.000000000000000000, 0.000000000000000000, -186.0000000000000000 ) ) ;
#13348=FACE_BOUND ( 'NONE', #4195, .T. ) ;
#13359=AXIS2_PLACEMENT_3D ( 'NONE', #655, #13944, #7198 ) ;
#13362=MECHANICAL_DESIGN_GEOMETRIC_PRESENTATION_REPRESENTATION('',(#12667),#12679);
#13394=PRODUCT ( 'roller', 'roller', '', ( #1739 ) ) ;
#13401=EDGE_CURVE ( 'NONE', #7342, #8845, #7364, .T. ) ;
#13419=CARTESIAN_POINT ( 'NONE',  ( 20.00000000000000000, 2.449293598294706513E-15, 190.0000000000000000 ) ) ;
#13422=CARTESIAN_POINT ( 'NONE',  ( 12.00000000000000000, 1.469576158976823947E-15, 190.0000000000000000 ) ) ;
#13439=CARTESIAN_POINT ( 'NONE',  ( 0.000000000000000000, 0.000000000000000000, -190.0000000000000000 ) ) ;
#13475=FACE_OUTER_BOUND ( 'NONE', #11340, .T. ) ;
#13483=MECHANICAL_DESIGN_GEOMETRIC_PRESENTATION_REPRESENTATION('',(#4003),#491);
#13536=CARTESIAN_POINT ( 'NONE',  ( -13.50000000000000000, 1.653273178848926867E-15, 190.0000000000000000 ) ) ;
#13591=VECTOR ( 'NONE', #7627, 1000.000000000000000 ) ;
#13595=CIRCLE ( 'NONE', #11521, 12.00000000000000000 ) ;
#13740=SURFACE_SIDE_STYLE ('',( #1620 ) ) ;
#13790=EDGE_LOOP ( 'NONE', ( #3885, #456, #12463, #9486 ) ) ;
#13813=EDGE_CURVE ( 'NONE', #7250, #6282, #3642, .T. ) ;
#13836=DIRECTION ( 'NONE',  ( 0.000000000000000000, 0.000000000000000000, 1.000000000000000000 ) ) ;
#13851=ORIENTED_EDGE ( 'NONE', *, *, #14017, .T. ) ;
#13875=CARTESIAN_POINT ( 'NONE',  ( 0.000000000000000000, 0.000000000000000000, 190.0000000000000000 ) ) ;
#13914=ORIENTED_EDGE ( 'NONE', *, *, #4202, .F. ) ;
#13916=DIRECTION ( 'NONE',  ( -1.000000000000000000, 0.000000000000000000, 0.000000000000000000 ) ) ;
#13941=ORIENTED_EDGE ( 'NONE', *, *, #4992, .T. ) ;
#13942=CARTESIAN_POINT ( 'NONE',  ( 0.000000000000000000, 0.000000000000000000, -190.0000000000000000 ) ) ;
#13944=DIRECTION ( 'NONE',  ( -0.000000000000000000, -0.000000000000000000, 1.000000000000000000 ) ) ;
#13962=DIRECTION ( 'NONE',  ( -0.000000000000000000, -0.000000000000000000, 1.000000000000000000 ) ) ;
#13971=CARTESIAN_POINT ( 'NONE',  ( 0.000000000000000000, 0.000000000000000000, -186.0000000000000000 ) ) ;
#14017=EDGE_CURVE ( 'NONE', #6282, #7250, #4123, .T. ) ;
#14030=ORIENTED_EDGE ( 'NONE', *, *, #1331, .T. ) ;
#14039=AXIS2_PLACEMENT_3D ( 'NONE', #10508, #9418, #5077 ) ;
#14105=AXIS2_PLACEMENT_3D ( 'NONE', #12545, #11319, #12609 ) ;
#14226=CARTESIAN_POINT ( 'NONE',  ( 0.000000000000000000, 0.000000000000000000, -186.0000000000000000 ) ) ;
#14397=COLOUR_RGB('Sky Blue',0.24,0.69,0.87);
#14398=FILL_AREA_STYLE_COLOUR('',#14397);
#14399=FILL_AREA_STYLE('',(#14398));
#14400=SURFACE_STYLE_FILL_AREA(#14399);
#14401=SURFACE_SIDE_STYLE('',(#14400));
#14402=SURFACE_STYLE_USAGE(.BOTH.,#14401);
#14403=PRESENTATION_STYLE_ASSIGNMENT((#14402));
ENDSEC;
END-ISO-10303-21;
